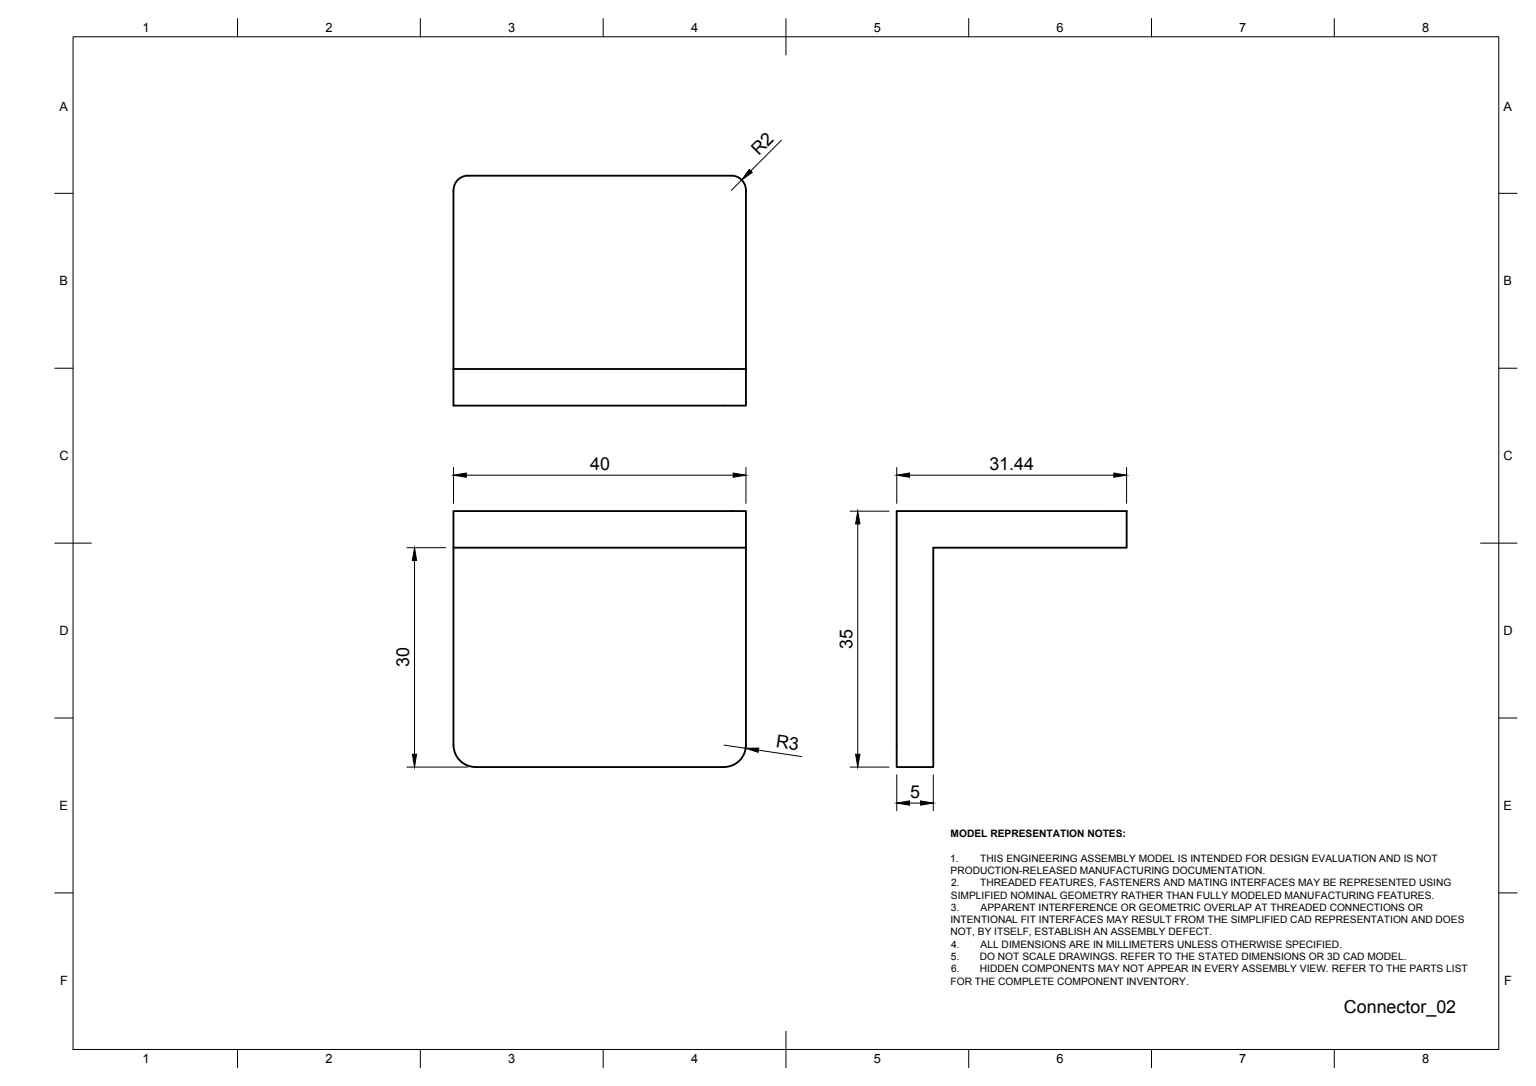
ISO-10303-21;
HEADER;
/* Generated by software containing ST-Developer
 * from STEP Tools, Inc. (www.steptools.com) 
 */

FILE_DESCRIPTION(
/* description */ (''),
/* implementation_level */ '2;1');

FILE_NAME(
/* name */ 'Connector_02.step',
/* time_stamp */ '2026-10-05T19:45:59-07:00',
/* author */ (''),
/* organization */ (''),
/* preprocessor_version */ 'ST-DEVELOPER v20.2',
/* originating_system */ 'Autodesk Translation Framework v15.15.0.0',
/* authorisation */ '');

FILE_SCHEMA (('AUTOMOTIVE_DESIGN { 1 0 10303 214 3 1 1 }'));
ENDSEC;

DATA;
#10=MECHANICAL_DESIGN_GEOMETRIC_PRESENTATION_REPRESENTATION('',(#97),#2462);
#79=SHAPE_REPRESENTATION_RELATIONSHIP('SRR','None',#2505,#88);
#88=ADVANCED_BREP_SHAPE_REPRESENTATION('',(#106),#2460);
#97=STYLED_ITEM('',(#2552),#106);
#106=MANIFOLD_SOLID_BREP('Body1',#1334);
#142=PLANE('',#1527);
#143=PLANE('',#1528);
#144=PLANE('',#1532);
#145=PLANE('',#1536);
#146=PLANE('',#1538);
#147=PLANE('',#1541);
#148=PLANE('',#1542);
#149=PLANE('',#1543);
#215=FACE_OUTER_BOUND('',#308,.T.);
#216=FACE_OUTER_BOUND('',#309,.T.);
#217=FACE_OUTER_BOUND('',#310,.T.);
#218=FACE_OUTER_BOUND('',#311,.T.);
#219=FACE_OUTER_BOUND('',#312,.T.);
#220=FACE_OUTER_BOUND('',#313,.T.);
#221=FACE_OUTER_BOUND('',#314,.T.);
#222=FACE_OUTER_BOUND('',#315,.T.);
#223=FACE_OUTER_BOUND('',#316,.T.);
#224=FACE_OUTER_BOUND('',#317,.T.);
#225=FACE_OUTER_BOUND('',#318,.T.);
#226=FACE_OUTER_BOUND('',#319,.T.);
#308=EDGE_LOOP('',(#1102,#1103,#1104,#1105));
#309=EDGE_LOOP('',(#1106,#1107,#1108,#1109));
#310=EDGE_LOOP('',(#1110,#1111,#1112,#1113,#1114,#1115));
#311=EDGE_LOOP('',(#1116,#1117,#1118,#1119));
#312=EDGE_LOOP('',(#1120,#1121,#1122,#1123,#1124,#1125));
#313=EDGE_LOOP('',(#1126,#1127,#1128,#1129));
#314=EDGE_LOOP('',(#1130,#1131,#1132,#1133,#1134,#1135));
#315=EDGE_LOOP('',(#1136,#1137,#1138,#1139));
#316=EDGE_LOOP('',(#1140,#1141,#1142,#1143));
#317=EDGE_LOOP('',(#1144,#1145,#1146,#1147,#1148,#1149));
#318=EDGE_LOOP('',(#1150,#1151,#1152,#1153,#1154,#1155));
#319=EDGE_LOOP('',(#1156,#1157,#1158,#1159,#1160,#1161));
#411=LINE('',#2305,#530);
#412=LINE('',#2308,#531);
#413=LINE('',#2311,#532);
#414=LINE('',#2313,#533);
#415=LINE('',#2314,#534);
#416=LINE('',#2317,#535);
#417=LINE('',#2319,#536);
#418=LINE('',#2321,#537);
#419=LINE('',#2325,#538);
#420=LINE('',#2329,#539);
#421=LINE('',#2331,#540);
#422=LINE('',#2333,#541);
#423=LINE('',#2334,#542);
#424=LINE('',#2340,#543);
#425=LINE('',#2343,#544);
#426=LINE('',#2345,#545);
#427=LINE('',#2348,#546);
#428=LINE('',#2351,#547);
#429=LINE('',#2352,#548);
#430=LINE('',#2357,#549);
#431=LINE('',#2358,#550);
#432=LINE('',#2360,#551);
#530=VECTOR('',#1830,10.);
#531=VECTOR('',#1833,10.);
#532=VECTOR('',#1836,10.);
#533=VECTOR('',#1837,10.);
#534=VECTOR('',#1838,10.);
#535=VECTOR('',#1841,10.);
#536=VECTOR('',#1842,10.);
#537=VECTOR('',#1843,10.);
#538=VECTOR('',#1848,10.);
#539=VECTOR('',#1853,10.);
#540=VECTOR('',#1854,10.);
#541=VECTOR('',#1855,10.);
#542=VECTOR('',#1856,10.);
#543=VECTOR('',#1861,10.);
#544=VECTOR('',#1864,10.);
#545=VECTOR('',#1867,10.);
#546=VECTOR('',#1870,10.);
#547=VECTOR('',#1873,10.);
#548=VECTOR('',#1874,10.);
#549=VECTOR('',#1881,10.);
#550=VECTOR('',#1882,10.);
#551=VECTOR('',#1885,10.);
#607=CIRCLE('',#1525,2.);
#608=CIRCLE('',#1526,2.);
#609=CIRCLE('',#1529,2.);
#610=CIRCLE('',#1531,2.);
#611=CIRCLE('',#1534,3.);
#612=CIRCLE('',#1535,3.);
#613=CIRCLE('',#1537,3.);
#614=CIRCLE('',#1540,3.);
#690=VERTEX_POINT('',#2301);
#691=VERTEX_POINT('',#2302);
#692=VERTEX_POINT('',#2304);
#693=VERTEX_POINT('',#2306);
#694=VERTEX_POINT('',#2310);
#695=VERTEX_POINT('',#2312);
#696=VERTEX_POINT('',#2316);
#697=VERTEX_POINT('',#2318);
#698=VERTEX_POINT('',#2320);
#699=VERTEX_POINT('',#2324);
#700=VERTEX_POINT('',#2328);
#701=VERTEX_POINT('',#2330);
#702=VERTEX_POINT('',#2332);
#703=VERTEX_POINT('',#2336);
#704=VERTEX_POINT('',#2337);
#705=VERTEX_POINT('',#2339);
#706=VERTEX_POINT('',#2341);
#707=VERTEX_POINT('',#2346);
#708=VERTEX_POINT('',#2350);
#709=VERTEX_POINT('',#2356);
#832=EDGE_CURVE('',#690,#691,#607,.T.);
#833=EDGE_CURVE('',#691,#692,#411,.T.);
#834=EDGE_CURVE('',#692,#693,#608,.T.);
#835=EDGE_CURVE('',#693,#690,#412,.T.);
#836=EDGE_CURVE('',#694,#693,#413,.T.);
#837=EDGE_CURVE('',#695,#694,#414,.T.);
#838=EDGE_CURVE('',#690,#695,#415,.T.);
#839=EDGE_CURVE('',#696,#692,#416,.T.);
#840=EDGE_CURVE('',#696,#697,#417,.T.);
#841=EDGE_CURVE('',#698,#697,#418,.T.);
#842=EDGE_CURVE('',#694,#698,#609,.T.);
#843=EDGE_CURVE('',#698,#699,#419,.T.);
#844=EDGE_CURVE('',#699,#695,#610,.T.);
#845=EDGE_CURVE('',#700,#691,#420,.T.);
#846=EDGE_CURVE('',#700,#701,#421,.T.);
#847=EDGE_CURVE('',#701,#702,#422,.T.);
#848=EDGE_CURVE('',#696,#702,#423,.T.);
#849=EDGE_CURVE('',#703,#704,#611,.T.);
#850=EDGE_CURVE('',#705,#703,#424,.T.);
#851=EDGE_CURVE('',#706,#705,#612,.T.);
#852=EDGE_CURVE('',#704,#706,#425,.T.);
#853=EDGE_CURVE('',#697,#705,#426,.T.);
#854=EDGE_CURVE('',#702,#707,#613,.T.);
#855=EDGE_CURVE('',#707,#706,#427,.T.);
#856=EDGE_CURVE('',#707,#708,#428,.T.);
#857=EDGE_CURVE('',#704,#708,#429,.T.);
#858=EDGE_CURVE('',#708,#701,#614,.T.);
#859=EDGE_CURVE('',#699,#709,#430,.T.);
#860=EDGE_CURVE('',#709,#700,#431,.T.);
#861=EDGE_CURVE('',#709,#703,#432,.T.);
#1102=ORIENTED_EDGE('',*,*,#832,.T.);
#1103=ORIENTED_EDGE('',*,*,#833,.T.);
#1104=ORIENTED_EDGE('',*,*,#834,.T.);
#1105=ORIENTED_EDGE('',*,*,#835,.T.);
#1106=ORIENTED_EDGE('',*,*,#835,.F.);
#1107=ORIENTED_EDGE('',*,*,#836,.F.);
#1108=ORIENTED_EDGE('',*,*,#837,.F.);
#1109=ORIENTED_EDGE('',*,*,#838,.F.);
#1110=ORIENTED_EDGE('',*,*,#834,.F.);
#1111=ORIENTED_EDGE('',*,*,#839,.F.);
#1112=ORIENTED_EDGE('',*,*,#840,.T.);
#1113=ORIENTED_EDGE('',*,*,#841,.F.);
#1114=ORIENTED_EDGE('',*,*,#842,.F.);
#1115=ORIENTED_EDGE('',*,*,#836,.T.);
#1116=ORIENTED_EDGE('',*,*,#842,.T.);
#1117=ORIENTED_EDGE('',*,*,#843,.T.);
#1118=ORIENTED_EDGE('',*,*,#844,.T.);
#1119=ORIENTED_EDGE('',*,*,#837,.T.);
#1120=ORIENTED_EDGE('',*,*,#833,.F.);
#1121=ORIENTED_EDGE('',*,*,#845,.F.);
#1122=ORIENTED_EDGE('',*,*,#846,.T.);
#1123=ORIENTED_EDGE('',*,*,#847,.T.);
#1124=ORIENTED_EDGE('',*,*,#848,.F.);
#1125=ORIENTED_EDGE('',*,*,#839,.T.);
#1126=ORIENTED_EDGE('',*,*,#849,.F.);
#1127=ORIENTED_EDGE('',*,*,#850,.F.);
#1128=ORIENTED_EDGE('',*,*,#851,.F.);
#1129=ORIENTED_EDGE('',*,*,#852,.F.);
#1130=ORIENTED_EDGE('',*,*,#851,.T.);
#1131=ORIENTED_EDGE('',*,*,#853,.F.);
#1132=ORIENTED_EDGE('',*,*,#840,.F.);
#1133=ORIENTED_EDGE('',*,*,#848,.T.);
#1134=ORIENTED_EDGE('',*,*,#854,.T.);
#1135=ORIENTED_EDGE('',*,*,#855,.T.);
#1136=ORIENTED_EDGE('',*,*,#852,.T.);
#1137=ORIENTED_EDGE('',*,*,#855,.F.);
#1138=ORIENTED_EDGE('',*,*,#856,.T.);
#1139=ORIENTED_EDGE('',*,*,#857,.F.);
#1140=ORIENTED_EDGE('',*,*,#854,.F.);
#1141=ORIENTED_EDGE('',*,*,#847,.F.);
#1142=ORIENTED_EDGE('',*,*,#858,.F.);
#1143=ORIENTED_EDGE('',*,*,#856,.F.);
#1144=ORIENTED_EDGE('',*,*,#832,.F.);
#1145=ORIENTED_EDGE('',*,*,#838,.T.);
#1146=ORIENTED_EDGE('',*,*,#844,.F.);
#1147=ORIENTED_EDGE('',*,*,#859,.T.);
#1148=ORIENTED_EDGE('',*,*,#860,.T.);
#1149=ORIENTED_EDGE('',*,*,#845,.T.);
#1150=ORIENTED_EDGE('',*,*,#849,.T.);
#1151=ORIENTED_EDGE('',*,*,#857,.T.);
#1152=ORIENTED_EDGE('',*,*,#858,.T.);
#1153=ORIENTED_EDGE('',*,*,#846,.F.);
#1154=ORIENTED_EDGE('',*,*,#860,.F.);
#1155=ORIENTED_EDGE('',*,*,#861,.T.);
#1156=ORIENTED_EDGE('',*,*,#843,.F.);
#1157=ORIENTED_EDGE('',*,*,#841,.T.);
#1158=ORIENTED_EDGE('',*,*,#853,.T.);
#1159=ORIENTED_EDGE('',*,*,#850,.T.);
#1160=ORIENTED_EDGE('',*,*,#861,.F.);
#1161=ORIENTED_EDGE('',*,*,#859,.F.);
#1241=CYLINDRICAL_SURFACE('',#1524,2.);
#1242=CYLINDRICAL_SURFACE('',#1530,2.);
#1243=CYLINDRICAL_SURFACE('',#1533,3.);
#1244=CYLINDRICAL_SURFACE('',#1539,3.);
#1297=ADVANCED_FACE('',(#215),#1241,.T.);
#1298=ADVANCED_FACE('',(#216),#142,.F.);
#1299=ADVANCED_FACE('',(#217),#143,.F.);
#1300=ADVANCED_FACE('',(#218),#1242,.T.);
#1301=ADVANCED_FACE('',(#219),#144,.F.);
#1302=ADVANCED_FACE('',(#220),#1243,.T.);
#1303=ADVANCED_FACE('',(#221),#145,.F.);
#1304=ADVANCED_FACE('',(#222),#146,.F.);
#1305=ADVANCED_FACE('',(#223),#1244,.T.);
#1306=ADVANCED_FACE('',(#224),#147,.T.);
#1307=ADVANCED_FACE('',(#225),#148,.F.);
#1308=ADVANCED_FACE('',(#226),#149,.F.);
#1334=CLOSED_SHELL('',(#1297,#1298,#1299,#1300,#1301,#1302,#1303,#1304,
#1305,#1306,#1307,#1308));
#1523=AXIS2_PLACEMENT_3D('',#2299,#1824,#1825);
#1524=AXIS2_PLACEMENT_3D('',#2300,#1826,#1827);
#1525=AXIS2_PLACEMENT_3D('',#2303,#1828,#1829);
#1526=AXIS2_PLACEMENT_3D('',#2307,#1831,#1832);
#1527=AXIS2_PLACEMENT_3D('',#2309,#1834,#1835);
#1528=AXIS2_PLACEMENT_3D('',#2315,#1839,#1840);
#1529=AXIS2_PLACEMENT_3D('',#2322,#1844,#1845);
#1530=AXIS2_PLACEMENT_3D('',#2323,#1846,#1847);
#1531=AXIS2_PLACEMENT_3D('',#2326,#1849,#1850);
#1532=AXIS2_PLACEMENT_3D('',#2327,#1851,#1852);
#1533=AXIS2_PLACEMENT_3D('',#2335,#1857,#1858);
#1534=AXIS2_PLACEMENT_3D('',#2338,#1859,#1860);
#1535=AXIS2_PLACEMENT_3D('',#2342,#1862,#1863);
#1536=AXIS2_PLACEMENT_3D('',#2344,#1865,#1866);
#1537=AXIS2_PLACEMENT_3D('',#2347,#1868,#1869);
#1538=AXIS2_PLACEMENT_3D('',#2349,#1871,#1872);
#1539=AXIS2_PLACEMENT_3D('',#2353,#1875,#1876);
#1540=AXIS2_PLACEMENT_3D('',#2354,#1877,#1878);
#1541=AXIS2_PLACEMENT_3D('',#2355,#1879,#1880);
#1542=AXIS2_PLACEMENT_3D('',#2359,#1883,#1884);
#1543=AXIS2_PLACEMENT_3D('',#2361,#1886,#1887);
#1824=DIRECTION('axis',(0.,0.,1.));
#1825=DIRECTION('refdir',(1.,0.,0.));
#1826=DIRECTION('center_axis',(1.,0.,0.));
#1827=DIRECTION('ref_axis',(0.,0.707106781186548,0.707106781186547));
#1828=DIRECTION('center_axis',(-1.,0.,0.));
#1829=DIRECTION('ref_axis',(0.,0.707106781186548,0.707106781186547));
#1830=DIRECTION('',(-1.,0.,0.));
#1831=DIRECTION('center_axis',(1.,0.,0.));
#1832=DIRECTION('ref_axis',(0.,0.707106781186548,0.707106781186547));
#1833=DIRECTION('',(1.,0.,0.));
#1834=DIRECTION('center_axis',(0.,0.,-1.));
#1835=DIRECTION('ref_axis',(-1.,0.,0.));
#1836=DIRECTION('',(0.,1.,0.));
#1837=DIRECTION('',(-1.,0.,0.));
#1838=DIRECTION('',(0.,-1.,0.));
#1839=DIRECTION('center_axis',(1.,0.,0.));
#1840=DIRECTION('ref_axis',(0.,0.,-1.));
#1841=DIRECTION('',(0.,0.,1.));
#1842=DIRECTION('',(0.,-1.,0.));
#1843=DIRECTION('',(0.,0.,-1.));
#1844=DIRECTION('center_axis',(1.,0.,0.));
#1845=DIRECTION('ref_axis',(0.,-0.707106781186548,0.707106781186547));
#1846=DIRECTION('center_axis',(-1.,0.,0.));
#1847=DIRECTION('ref_axis',(0.,-0.707106781186548,0.707106781186547));
#1848=DIRECTION('',(1.,0.,0.));
#1849=DIRECTION('center_axis',(-1.,0.,0.));
#1850=DIRECTION('ref_axis',(0.,-0.707106781186548,0.707106781186547));
#1851=DIRECTION('center_axis',(0.,-1.,0.));
#1852=DIRECTION('ref_axis',(0.,0.,1.));
#1853=DIRECTION('',(0.,0.,1.));
#1854=DIRECTION('',(-1.,0.,0.));
#1855=DIRECTION('',(0.,0.,1.));
#1856=DIRECTION('',(-1.,0.,0.));
#1857=DIRECTION('center_axis',(0.,0.,1.));
#1858=DIRECTION('ref_axis',(-0.707106781186544,-0.707106781186551,0.));
#1859=DIRECTION('center_axis',(0.,0.,-1.));
#1860=DIRECTION('ref_axis',(-0.707106781186544,-0.707106781186551,0.));
#1861=DIRECTION('',(0.,0.,-1.));
#1862=DIRECTION('center_axis',(0.,0.,1.));
#1863=DIRECTION('ref_axis',(-0.707106781186544,-0.707106781186551,0.));
#1864=DIRECTION('',(0.,0.,1.));
#1865=DIRECTION('center_axis',(0.,0.,-1.));
#1866=DIRECTION('ref_axis',(0.,-1.,0.));
#1867=DIRECTION('',(-1.,0.,0.));
#1868=DIRECTION('center_axis',(0.,0.,1.));
#1869=DIRECTION('ref_axis',(-0.707106781186544,0.707106781186551,0.));
#1870=DIRECTION('',(0.,-1.,0.));
#1871=DIRECTION('center_axis',(1.,0.,0.));
#1872=DIRECTION('ref_axis',(0.,0.,-1.));
#1873=DIRECTION('',(0.,0.,-1.));
#1874=DIRECTION('',(0.,1.,0.));
#1875=DIRECTION('center_axis',(0.,0.,-1.));
#1876=DIRECTION('ref_axis',(-0.707106781186544,0.707106781186551,0.));
#1877=DIRECTION('center_axis',(0.,0.,-1.));
#1878=DIRECTION('ref_axis',(-0.707106781186544,0.707106781186551,0.));
#1879=DIRECTION('center_axis',(1.,0.,0.));
#1880=DIRECTION('ref_axis',(0.,1.,0.));
#1881=DIRECTION('',(0.,0.,-1.));
#1882=DIRECTION('',(0.,1.,0.));
#1883=DIRECTION('center_axis',(0.,0.,1.));
#1884=DIRECTION('ref_axis',(0.,1.,0.));
#1885=DIRECTION('',(-1.,0.,0.));
#1886=DIRECTION('center_axis',(0.,1.,0.));
#1887=DIRECTION('ref_axis',(0.,0.,-1.));
#2299=CARTESIAN_POINT('',(0.,0.,0.));
#2300=CARTESIAN_POINT('Origin',(0.,18.,9.43656992056115));
#2301=CARTESIAN_POINT('',(0.,18.,11.4365699205612));
#2302=CARTESIAN_POINT('',(0.,20.,9.43656992056115));
#2303=CARTESIAN_POINT('Origin',(0.,18.,9.43656992056115));
#2304=CARTESIAN_POINT('',(-5.,20.,9.43656992056115));
#2305=CARTESIAN_POINT('',(0.,20.,9.43656992056115));
#2306=CARTESIAN_POINT('',(-5.,18.,11.4365699205612));
#2307=CARTESIAN_POINT('Origin',(-5.,18.,9.43656992056115));
#2308=CARTESIAN_POINT('',(0.,18.,11.4365699205612));
#2309=CARTESIAN_POINT('Origin',(0.,-20.,11.4365699205612));
#2310=CARTESIAN_POINT('',(-5.,-18.,11.4365699205612));
#2311=CARTESIAN_POINT('',(-5.,-10.,11.4365699205612));
#2312=CARTESIAN_POINT('',(0.,-18.,11.4365699205612));
#2313=CARTESIAN_POINT('',(0.,-18.,11.4365699205612));
#2314=CARTESIAN_POINT('',(0.,-10.,11.4365699205612));
#2315=CARTESIAN_POINT('Origin',(-5.,0.,2.5));
#2316=CARTESIAN_POINT('',(-5.,20.,-15.));
#2317=CARTESIAN_POINT('',(-5.,20.,20.));
#2318=CARTESIAN_POINT('',(-5.,-20.,-15.));
#2319=CARTESIAN_POINT('',(-5.,10.,-15.));
#2320=CARTESIAN_POINT('',(-5.,-20.,9.43656992056115));
#2321=CARTESIAN_POINT('',(-5.,-20.,-20.));
#2322=CARTESIAN_POINT('Origin',(-5.,-18.,9.43656992056115));
#2323=CARTESIAN_POINT('Origin',(0.,-18.,9.43656992056115));
#2324=CARTESIAN_POINT('',(0.,-20.,9.43656992056115));
#2325=CARTESIAN_POINT('',(0.,-20.,9.43656992056115));
#2326=CARTESIAN_POINT('Origin',(0.,-18.,9.43656992056115));
#2327=CARTESIAN_POINT('Origin',(0.,20.,-20.));
#2328=CARTESIAN_POINT('',(0.,20.,-20.));
#2329=CARTESIAN_POINT('',(0.,20.,-20.));
#2330=CARTESIAN_POINT('',(-32.0000000000001,20.,-20.));
#2331=CARTESIAN_POINT('',(0.,20.,-20.));
#2332=CARTESIAN_POINT('',(-32.0000000000001,20.,-15.));
#2333=CARTESIAN_POINT('',(-32.0000000000001,20.,-18.75));
#2334=CARTESIAN_POINT('',(0.,20.,-15.));
#2335=CARTESIAN_POINT('Origin',(-32.0000000000001,-17.,-16.25));
#2336=CARTESIAN_POINT('',(-32.0000000000001,-20.,-20.));
#2337=CARTESIAN_POINT('',(-35.,-17.,-20.));
#2338=CARTESIAN_POINT('Origin',(-32.0000000000001,-17.,-20.));
#2339=CARTESIAN_POINT('',(-32.0000000000001,-20.,-15.));
#2340=CARTESIAN_POINT('',(-32.0000000000001,-20.,-16.25));
#2341=CARTESIAN_POINT('',(-35.,-17.,-15.));
#2342=CARTESIAN_POINT('Origin',(-32.0000000000001,-17.,-15.));
#2343=CARTESIAN_POINT('',(-35.,-17.,-16.25));
#2344=CARTESIAN_POINT('Origin',(0.,20.,-15.));
#2345=CARTESIAN_POINT('',(0.,-20.,-15.));
#2346=CARTESIAN_POINT('',(-35.,17.,-15.));
#2347=CARTESIAN_POINT('Origin',(-32.0000000000001,17.,-15.));
#2348=CARTESIAN_POINT('',(-35.,20.,-15.));
#2349=CARTESIAN_POINT('Origin',(-35.,0.,-17.5));
#2350=CARTESIAN_POINT('',(-35.,17.,-20.));
#2351=CARTESIAN_POINT('',(-35.,17.,-18.75));
#2352=CARTESIAN_POINT('',(-35.,-20.,-20.));
#2353=CARTESIAN_POINT('Origin',(-32.0000000000001,17.,-18.75));
#2354=CARTESIAN_POINT('Origin',(-32.0000000000001,17.,-20.));
#2355=CARTESIAN_POINT('Origin',(0.,0.,-17.5));
#2356=CARTESIAN_POINT('',(0.,-20.,-20.));
#2357=CARTESIAN_POINT('',(0.,-20.,-15.));
#2358=CARTESIAN_POINT('',(0.,-20.,-20.));
#2359=CARTESIAN_POINT('Origin',(0.,-20.,-20.));
#2360=CARTESIAN_POINT('',(0.,-20.,-20.));
#2361=CARTESIAN_POINT('Origin',(0.,-20.,-15.));
#2449=UNCERTAINTY_MEASURE_WITH_UNIT(LENGTH_MEASURE(0.01),#2463,
'DISTANCE_ACCURACY_VALUE',
'Maximum model space distance between geometric entities at asserted c
onnectivities');
#2451=UNCERTAINTY_MEASURE_WITH_UNIT(LENGTH_MEASURE(0.01),#2463,
'DISTANCE_ACCURACY_VALUE',
'Maximum model space distance between geometric entities at asserted c
onnectivities');
#2460=(
GEOMETRIC_REPRESENTATION_CONTEXT(3)
GLOBAL_UNCERTAINTY_ASSIGNED_CONTEXT((#2449))
GLOBAL_UNIT_ASSIGNED_CONTEXT((#2463,#2465,#2466))
REPRESENTATION_CONTEXT('','3D')
);
#2462=(
GEOMETRIC_REPRESENTATION_CONTEXT(3)
GLOBAL_UNCERTAINTY_ASSIGNED_CONTEXT((#2451))
GLOBAL_UNIT_ASSIGNED_CONTEXT((#2463,#2465,#2466))
REPRESENTATION_CONTEXT('','3D')
);
#2463=(
LENGTH_UNIT()
NAMED_UNIT(*)
SI_UNIT(.MILLI.,.METRE.)
);
#2465=(
NAMED_UNIT(*)
PLANE_ANGLE_UNIT()
SI_UNIT($,.RADIAN.)
);
#2466=(
NAMED_UNIT(*)
SI_UNIT($,.STERADIAN.)
SOLID_ANGLE_UNIT()
);
#2475=SHAPE_DEFINITION_REPRESENTATION(#2485,#2505);
#2485=PRODUCT_DEFINITION_SHAPE('',$,#2516);
#2505=SHAPE_REPRESENTATION('',(#1523),#2460);
#2507=PRODUCT_DEFINITION_CONTEXT('part definition',#2539,'design');
#2516=PRODUCT_DEFINITION('Connector_02','Connector_02',#2526,#2507);
#2526=PRODUCT_DEFINITION_FORMATION('',$,#2549);
#2539=APPLICATION_CONTEXT(
'Core Data for Automotive Mechanical Design Process');
#2540=PRODUCT_CONTEXT('part definition',#2539,'mechanical');
#2549=PRODUCT('Connector_02','Connector_02',$,(#2540));
#2552=PRESENTATION_STYLE_ASSIGNMENT((#2555));
#2555=SURFACE_STYLE_USAGE(.BOTH.,#2558);
#2558=SURFACE_SIDE_STYLE('',(#2561));
#2561=SURFACE_STYLE_FILL_AREA(#2564);
#2564=FILL_AREA_STYLE('Opaque(160,160,160)',(#2567));
#2567=FILL_AREA_STYLE_COLOUR('Opaque(160,160,160)',#2570);
#2570=COLOUR_RGB('Opaque(160,160,160)', 0.09019608, 0.27058824, 0.51372549);
ENDSEC;
END-ISO-10303-21;
